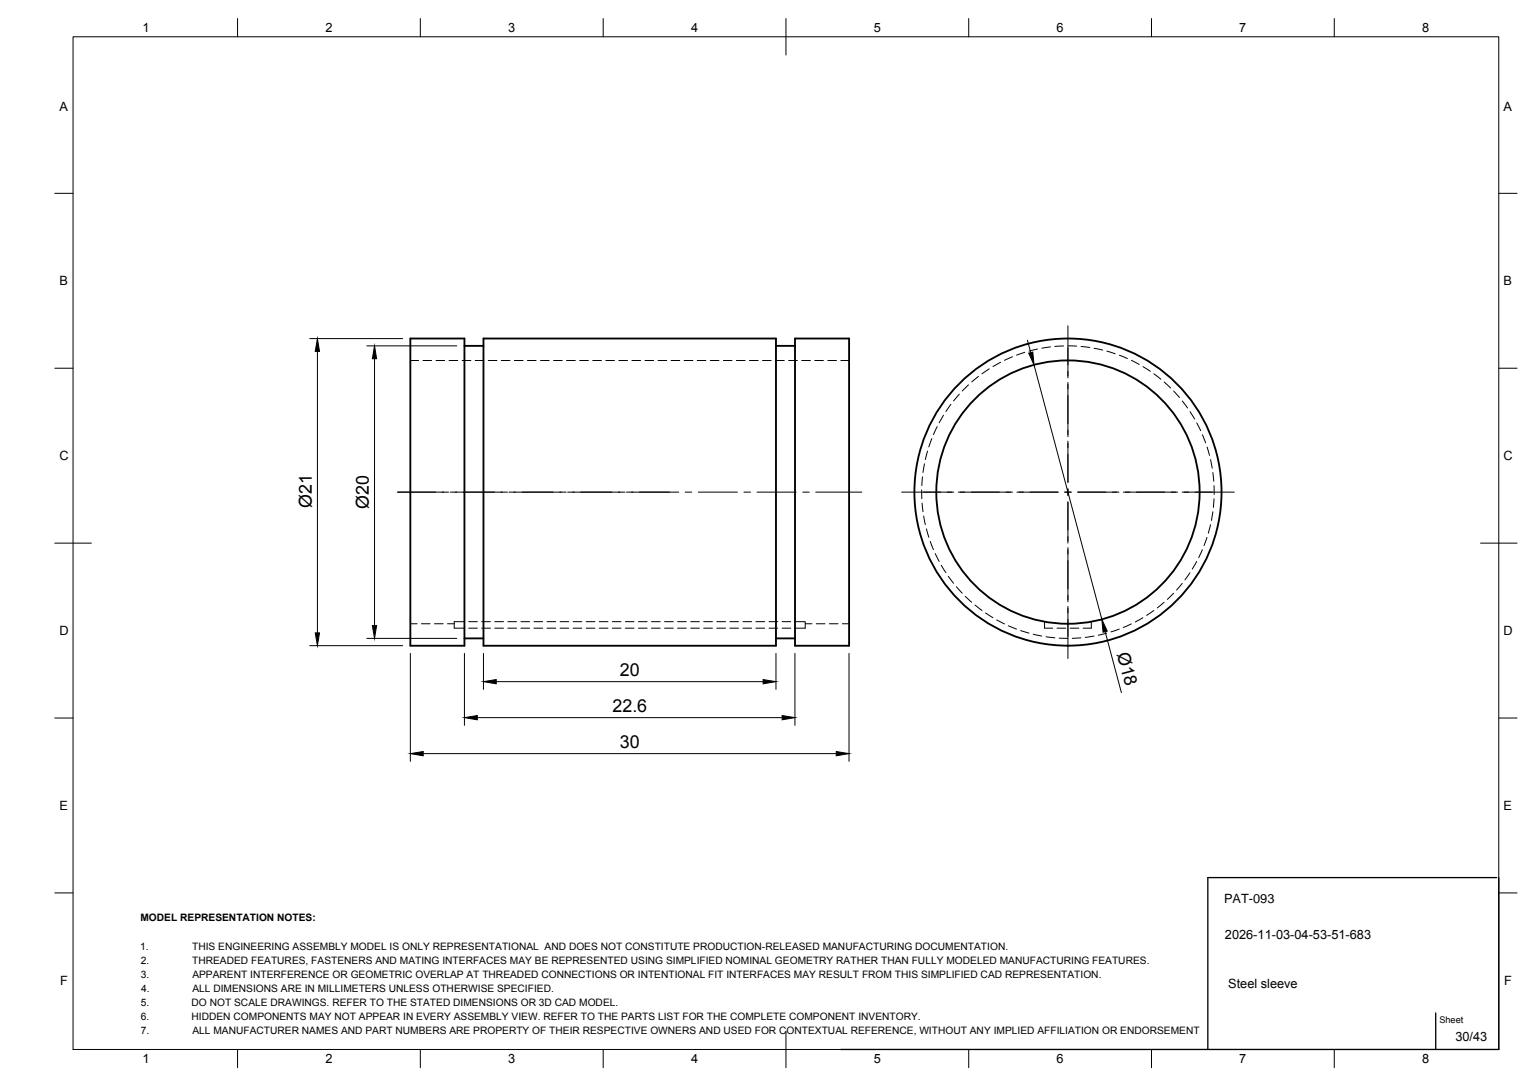
ISO-10303-21;
HEADER;
/* Generated by software containing ST-Developer
 * from STEP Tools, Inc. (www.steptools.com) 
 */

FILE_DESCRIPTION(
/* description */ ('Self-centering screw clamp'),
/* implementation_level */ '2;1');

FILE_NAME(
/* name */ 'Steel sleeve.step',
/* time_stamp */ '2026-10-28T03:25:31-07:00',
/* author */ (''),
/* organization */ (''),
/* preprocessor_version */ 'ST-DEVELOPER v20.2',
/* originating_system */ 'Autodesk Translation Framework v15.17.0.0',
/* authorisation */ '');

FILE_SCHEMA (('AUTOMOTIVE_DESIGN { 1 0 10303 214 3 1 1 }'));
ENDSEC;

DATA;
#10=MECHANICAL_DESIGN_GEOMETRIC_PRESENTATION_REPRESENTATION('',(#660),#16799);
#571=SHAPE_REPRESENTATION_RELATIONSHIP('SRR','None',#17048,#612);
#612=ADVANCED_BREP_SHAPE_REPRESENTATION('',(#708),#16786);
#660=STYLED_ITEM('',(#17340),#708);
#708=MANIFOLD_SOLID_BREP('Body1',#9111);
#981=FACE_BOUND('',#2433,.T.);
#982=FACE_BOUND('',#2436,.T.);
#983=FACE_BOUND('',#2439,.T.);
#984=FACE_BOUND('',#2442,.T.);
#985=FACE_BOUND('',#2445,.T.);
#986=FACE_BOUND('',#2448,.T.);
#987=FACE_BOUND('',#2450,.T.);
#1200=PLANE('',#10430);
#1201=PLANE('',#10432);
#1202=PLANE('',#10433);
#1203=PLANE('',#10435);
#1204=PLANE('',#10436);
#1205=PLANE('',#10437);
#1206=PLANE('',#10442);
#1207=PLANE('',#10446);
#1208=PLANE('',#10450);
#1209=PLANE('',#10454);
#1210=PLANE('',#10458);
#1660=FACE_OUTER_BOUND('',#2427,.T.);
#1661=FACE_OUTER_BOUND('',#2428,.T.);
#1662=FACE_OUTER_BOUND('',#2429,.T.);
#1663=FACE_OUTER_BOUND('',#2430,.T.);
#1664=FACE_OUTER_BOUND('',#2431,.T.);
#1665=FACE_OUTER_BOUND('',#2432,.T.);
#1666=FACE_OUTER_BOUND('',#2434,.T.);
#1667=FACE_OUTER_BOUND('',#2435,.T.);
#1668=FACE_OUTER_BOUND('',#2437,.T.);
#1669=FACE_OUTER_BOUND('',#2438,.T.);
#1670=FACE_OUTER_BOUND('',#2440,.T.);
#1671=FACE_OUTER_BOUND('',#2441,.T.);
#1672=FACE_OUTER_BOUND('',#2443,.T.);
#1673=FACE_OUTER_BOUND('',#2444,.T.);
#1674=FACE_OUTER_BOUND('',#2446,.T.);
#1675=FACE_OUTER_BOUND('',#2447,.T.);
#1676=FACE_OUTER_BOUND('',#2449,.T.);
#2427=EDGE_LOOP('',(#7911,#7912,#7913,#7914));
#2428=EDGE_LOOP('',(#7915,#7916,#7917,#7918));
#2429=EDGE_LOOP('',(#7919,#7920,#7921,#7922));
#2430=EDGE_LOOP('',(#7923,#7924,#7925,#7926));
#2431=EDGE_LOOP('',(#7927,#7928,#7929,#7930));
#2432=EDGE_LOOP('',(#7931));
#2433=EDGE_LOOP('',(#7932));
#2434=EDGE_LOOP('',(#7933,#7934,#7935,#7936));
#2435=EDGE_LOOP('',(#7937));
#2436=EDGE_LOOP('',(#7938));
#2437=EDGE_LOOP('',(#7939,#7940,#7941,#7942));
#2438=EDGE_LOOP('',(#7943));
#2439=EDGE_LOOP('',(#7944));
#2440=EDGE_LOOP('',(#7945,#7946,#7947,#7948));
#2441=EDGE_LOOP('',(#7949));
#2442=EDGE_LOOP('',(#7950));
#2443=EDGE_LOOP('',(#7951,#7952,#7953,#7954));
#2444=EDGE_LOOP('',(#7955));
#2445=EDGE_LOOP('',(#7956));
#2446=EDGE_LOOP('',(#7957,#7958,#7959,#7960));
#2447=EDGE_LOOP('',(#7961));
#2448=EDGE_LOOP('',(#7962));
#2449=EDGE_LOOP('',(#7963,#7964,#7965,#7966));
#2450=EDGE_LOOP('',(#7967,#7968,#7969,#7970));
#3026=LINE('',#15984,#3599);
#3027=LINE('',#15986,#3600);
#3028=LINE('',#15987,#3601);
#3029=LINE('',#15990,#3602);
#3030=LINE('',#15992,#3603);
#3031=LINE('',#15993,#3604);
#3032=LINE('',#15998,#3605);
#3033=LINE('',#15999,#3606);
#3034=LINE('',#16001,#3607);
#3035=LINE('',#16002,#3608);
#3036=LINE('',#16012,#3609);
#3037=LINE('',#16019,#3610);
#3038=LINE('',#16026,#3611);
#3039=LINE('',#16033,#3612);
#3040=LINE('',#16040,#3613);
#3041=LINE('',#16045,#3614);
#3599=VECTOR('',#12911,1.);
#3600=VECTOR('',#12912,1.);
#3601=VECTOR('',#12913,1.);
#3602=VECTOR('',#12916,1.);
#3603=VECTOR('',#12917,1.);
#3604=VECTOR('',#12918,1.);
#3605=VECTOR('',#12923,1.);
#3606=VECTOR('',#12924,1.);
#3607=VECTOR('',#12927,1.);
#3608=VECTOR('',#12928,1.);
#3609=VECTOR('',#12941,1.05);
#3610=VECTOR('',#12950,1.);
#3611=VECTOR('',#12959,1.05);
#3612=VECTOR('',#12968,1.);
#3613=VECTOR('',#12977,1.05);
#3614=VECTOR('',#12984,0.9);
#4148=CIRCLE('',#10431,0.9);
#4149=CIRCLE('',#10434,0.9);
#4150=CIRCLE('',#10438,1.05);
#4151=CIRCLE('',#10439,0.9);
#4152=CIRCLE('',#10441,1.05);
#4153=CIRCLE('',#10443,1.);
#4154=CIRCLE('',#10445,1.);
#4155=CIRCLE('',#10447,1.05);
#4156=CIRCLE('',#10449,1.05);
#4157=CIRCLE('',#10451,1.);
#4158=CIRCLE('',#10453,1.);
#4159=CIRCLE('',#10455,1.05);
#4160=CIRCLE('',#10457,1.05);
#4161=CIRCLE('',#10459,0.9);
#4831=VERTEX_POINT('',#15980);
#4832=VERTEX_POINT('',#15981);
#4833=VERTEX_POINT('',#15983);
#4834=VERTEX_POINT('',#15985);
#4835=VERTEX_POINT('',#15989);
#4836=VERTEX_POINT('',#15991);
#4837=VERTEX_POINT('',#15995);
#4838=VERTEX_POINT('',#15997);
#4839=VERTEX_POINT('',#16005);
#4840=VERTEX_POINT('',#16007);
#4841=VERTEX_POINT('',#16010);
#4842=VERTEX_POINT('',#16014);
#4843=VERTEX_POINT('',#16017);
#4844=VERTEX_POINT('',#16021);
#4845=VERTEX_POINT('',#16024);
#4846=VERTEX_POINT('',#16028);
#4847=VERTEX_POINT('',#16031);
#4848=VERTEX_POINT('',#16035);
#4849=VERTEX_POINT('',#16038);
#4850=VERTEX_POINT('',#16042);
#5880=EDGE_CURVE('',#4831,#4832,#4148,.T.);
#5881=EDGE_CURVE('',#4833,#4831,#3026,.T.);
#5882=EDGE_CURVE('',#4834,#4833,#3027,.T.);
#5883=EDGE_CURVE('',#4832,#4834,#3028,.T.);
#5884=EDGE_CURVE('',#4832,#4835,#3029,.T.);
#5885=EDGE_CURVE('',#4836,#4834,#3030,.T.);
#5886=EDGE_CURVE('',#4836,#4835,#3031,.T.);
#5887=EDGE_CURVE('',#4835,#4837,#4149,.T.);
#5888=EDGE_CURVE('',#4838,#4836,#3032,.T.);
#5889=EDGE_CURVE('',#4837,#4838,#3033,.T.);
#5890=EDGE_CURVE('',#4837,#4831,#3034,.T.);
#5891=EDGE_CURVE('',#4838,#4833,#3035,.T.);
#5892=EDGE_CURVE('',#4839,#4839,#4150,.T.);
#5893=EDGE_CURVE('',#4840,#4840,#4151,.T.);
#5894=EDGE_CURVE('',#4841,#4841,#4152,.T.);
#5895=EDGE_CURVE('',#4841,#4839,#3036,.T.);
#5896=EDGE_CURVE('',#4842,#4842,#4153,.T.);
#5897=EDGE_CURVE('',#4843,#4843,#4154,.T.);
#5898=EDGE_CURVE('',#4843,#4842,#3037,.T.);
#5899=EDGE_CURVE('',#4844,#4844,#4155,.T.);
#5900=EDGE_CURVE('',#4845,#4845,#4156,.T.);
#5901=EDGE_CURVE('',#4845,#4844,#3038,.T.);
#5902=EDGE_CURVE('',#4846,#4846,#4157,.T.);
#5903=EDGE_CURVE('',#4847,#4847,#4158,.T.);
#5904=EDGE_CURVE('',#4847,#4846,#3039,.T.);
#5905=EDGE_CURVE('',#4848,#4848,#4159,.T.);
#5906=EDGE_CURVE('',#4849,#4849,#4160,.T.);
#5907=EDGE_CURVE('',#4849,#4848,#3040,.T.);
#5908=EDGE_CURVE('',#4850,#4850,#4161,.T.);
#5909=EDGE_CURVE('',#4850,#4840,#3041,.T.);
#7911=ORIENTED_EDGE('',*,*,#5880,.F.);
#7912=ORIENTED_EDGE('',*,*,#5881,.F.);
#7913=ORIENTED_EDGE('',*,*,#5882,.F.);
#7914=ORIENTED_EDGE('',*,*,#5883,.F.);
#7915=ORIENTED_EDGE('',*,*,#5884,.F.);
#7916=ORIENTED_EDGE('',*,*,#5883,.T.);
#7917=ORIENTED_EDGE('',*,*,#5885,.F.);
#7918=ORIENTED_EDGE('',*,*,#5886,.T.);
#7919=ORIENTED_EDGE('',*,*,#5887,.F.);
#7920=ORIENTED_EDGE('',*,*,#5886,.F.);
#7921=ORIENTED_EDGE('',*,*,#5888,.F.);
#7922=ORIENTED_EDGE('',*,*,#5889,.F.);
#7923=ORIENTED_EDGE('',*,*,#5890,.F.);
#7924=ORIENTED_EDGE('',*,*,#5889,.T.);
#7925=ORIENTED_EDGE('',*,*,#5891,.T.);
#7926=ORIENTED_EDGE('',*,*,#5881,.T.);
#7927=ORIENTED_EDGE('',*,*,#5891,.F.);
#7928=ORIENTED_EDGE('',*,*,#5888,.T.);
#7929=ORIENTED_EDGE('',*,*,#5885,.T.);
#7930=ORIENTED_EDGE('',*,*,#5882,.T.);
#7931=ORIENTED_EDGE('',*,*,#5892,.F.);
#7932=ORIENTED_EDGE('',*,*,#5893,.T.);
#7933=ORIENTED_EDGE('',*,*,#5894,.F.);
#7934=ORIENTED_EDGE('',*,*,#5895,.T.);
#7935=ORIENTED_EDGE('',*,*,#5892,.T.);
#7936=ORIENTED_EDGE('',*,*,#5895,.F.);
#7937=ORIENTED_EDGE('',*,*,#5894,.T.);
#7938=ORIENTED_EDGE('',*,*,#5896,.F.);
#7939=ORIENTED_EDGE('',*,*,#5897,.F.);
#7940=ORIENTED_EDGE('',*,*,#5898,.T.);
#7941=ORIENTED_EDGE('',*,*,#5896,.T.);
#7942=ORIENTED_EDGE('',*,*,#5898,.F.);
#7943=ORIENTED_EDGE('',*,*,#5899,.F.);
#7944=ORIENTED_EDGE('',*,*,#5897,.T.);
#7945=ORIENTED_EDGE('',*,*,#5900,.F.);
#7946=ORIENTED_EDGE('',*,*,#5901,.T.);
#7947=ORIENTED_EDGE('',*,*,#5899,.T.);
#7948=ORIENTED_EDGE('',*,*,#5901,.F.);
#7949=ORIENTED_EDGE('',*,*,#5900,.T.);
#7950=ORIENTED_EDGE('',*,*,#5902,.F.);
#7951=ORIENTED_EDGE('',*,*,#5903,.F.);
#7952=ORIENTED_EDGE('',*,*,#5904,.T.);
#7953=ORIENTED_EDGE('',*,*,#5902,.T.);
#7954=ORIENTED_EDGE('',*,*,#5904,.F.);
#7955=ORIENTED_EDGE('',*,*,#5905,.F.);
#7956=ORIENTED_EDGE('',*,*,#5903,.T.);
#7957=ORIENTED_EDGE('',*,*,#5906,.F.);
#7958=ORIENTED_EDGE('',*,*,#5907,.T.);
#7959=ORIENTED_EDGE('',*,*,#5905,.T.);
#7960=ORIENTED_EDGE('',*,*,#5907,.F.);
#7961=ORIENTED_EDGE('',*,*,#5906,.T.);
#7962=ORIENTED_EDGE('',*,*,#5908,.F.);
#7963=ORIENTED_EDGE('',*,*,#5908,.T.);
#7964=ORIENTED_EDGE('',*,*,#5909,.T.);
#7965=ORIENTED_EDGE('',*,*,#5893,.F.);
#7966=ORIENTED_EDGE('',*,*,#5909,.F.);
#7967=ORIENTED_EDGE('',*,*,#5887,.T.);
#7968=ORIENTED_EDGE('',*,*,#5890,.T.);
#7969=ORIENTED_EDGE('',*,*,#5880,.T.);
#7970=ORIENTED_EDGE('',*,*,#5884,.T.);
#8536=CYLINDRICAL_SURFACE('',#10440,1.05);
#8537=CYLINDRICAL_SURFACE('',#10444,1.);
#8538=CYLINDRICAL_SURFACE('',#10448,1.05);
#8539=CYLINDRICAL_SURFACE('',#10452,1.);
#8540=CYLINDRICAL_SURFACE('',#10456,1.05);
#8541=CYLINDRICAL_SURFACE('',#10460,0.9);
#8958=ADVANCED_FACE('',(#1660),#1200,.F.);
#8959=ADVANCED_FACE('',(#1661),#1201,.F.);
#8960=ADVANCED_FACE('',(#1662),#1202,.F.);
#8961=ADVANCED_FACE('',(#1663),#1203,.F.);
#8962=ADVANCED_FACE('',(#1664),#1204,.F.);
#8963=ADVANCED_FACE('',(#1665,#981),#1205,.T.);
#8964=ADVANCED_FACE('',(#1666),#8536,.T.);
#8965=ADVANCED_FACE('',(#1667,#982),#1206,.T.);
#8966=ADVANCED_FACE('',(#1668),#8537,.T.);
#8967=ADVANCED_FACE('',(#1669,#983),#1207,.T.);
#8968=ADVANCED_FACE('',(#1670),#8538,.T.);
#8969=ADVANCED_FACE('',(#1671,#984),#1208,.T.);
#8970=ADVANCED_FACE('',(#1672),#8539,.T.);
#8971=ADVANCED_FACE('',(#1673,#985),#1209,.T.);
#8972=ADVANCED_FACE('',(#1674),#8540,.T.);
#8973=ADVANCED_FACE('',(#1675,#986),#1210,.T.);
#8974=ADVANCED_FACE('',(#1676,#987),#8541,.F.);
#9111=CLOSED_SHELL('',(#8958,#8959,#8960,#8961,#8962,#8963,#8964,#8965,
#8966,#8967,#8968,#8969,#8970,#8971,#8972,#8973,#8974));
#10429=AXIS2_PLACEMENT_3D('',#15978,#12905,#12906);
#10430=AXIS2_PLACEMENT_3D('',#15979,#12907,#12908);
#10431=AXIS2_PLACEMENT_3D('',#15982,#12909,#12910);
#10432=AXIS2_PLACEMENT_3D('',#15988,#12914,#12915);
#10433=AXIS2_PLACEMENT_3D('',#15994,#12919,#12920);
#10434=AXIS2_PLACEMENT_3D('',#15996,#12921,#12922);
#10435=AXIS2_PLACEMENT_3D('',#16000,#12925,#12926);
#10436=AXIS2_PLACEMENT_3D('',#16003,#12929,#12930);
#10437=AXIS2_PLACEMENT_3D('',#16004,#12931,#12932);
#10438=AXIS2_PLACEMENT_3D('',#16006,#12933,#12934);
#10439=AXIS2_PLACEMENT_3D('',#16008,#12935,#12936);
#10440=AXIS2_PLACEMENT_3D('',#16009,#12937,#12938);
#10441=AXIS2_PLACEMENT_3D('',#16011,#12939,#12940);
#10442=AXIS2_PLACEMENT_3D('',#16013,#12942,#12943);
#10443=AXIS2_PLACEMENT_3D('',#16015,#12944,#12945);
#10444=AXIS2_PLACEMENT_3D('',#16016,#12946,#12947);
#10445=AXIS2_PLACEMENT_3D('',#16018,#12948,#12949);
#10446=AXIS2_PLACEMENT_3D('',#16020,#12951,#12952);
#10447=AXIS2_PLACEMENT_3D('',#16022,#12953,#12954);
#10448=AXIS2_PLACEMENT_3D('',#16023,#12955,#12956);
#10449=AXIS2_PLACEMENT_3D('',#16025,#12957,#12958);
#10450=AXIS2_PLACEMENT_3D('',#16027,#12960,#12961);
#10451=AXIS2_PLACEMENT_3D('',#16029,#12962,#12963);
#10452=AXIS2_PLACEMENT_3D('',#16030,#12964,#12965);
#10453=AXIS2_PLACEMENT_3D('',#16032,#12966,#12967);
#10454=AXIS2_PLACEMENT_3D('',#16034,#12969,#12970);
#10455=AXIS2_PLACEMENT_3D('',#16036,#12971,#12972);
#10456=AXIS2_PLACEMENT_3D('',#16037,#12973,#12974);
#10457=AXIS2_PLACEMENT_3D('',#16039,#12975,#12976);
#10458=AXIS2_PLACEMENT_3D('',#16041,#12978,#12979);
#10459=AXIS2_PLACEMENT_3D('',#16043,#12980,#12981);
#10460=AXIS2_PLACEMENT_3D('',#16044,#12982,#12983);
#12905=DIRECTION('axis',(0.,0.,1.));
#12906=DIRECTION('refdir',(1.,0.,0.));
#12907=DIRECTION('center_axis',(0.,1.,0.));
#12908=DIRECTION('ref_axis',(0.,0.,1.));
#12909=DIRECTION('center_axis',(0.,-1.,0.));
#12910=DIRECTION('ref_axis',(1.,0.,0.));
#12911=DIRECTION('',(-1.,0.,0.));
#12912=DIRECTION('',(0.,0.,-1.));
#12913=DIRECTION('',(1.,0.,0.));
#12914=DIRECTION('center_axis',(0.,0.,1.));
#12915=DIRECTION('ref_axis',(1.,0.,0.));
#12916=DIRECTION('',(0.,-1.,0.));
#12917=DIRECTION('',(0.,1.,0.));
#12918=DIRECTION('',(-1.,0.,0.));
#12919=DIRECTION('center_axis',(0.,-1.,0.));
#12920=DIRECTION('ref_axis',(0.,0.,-1.));
#12921=DIRECTION('center_axis',(0.,1.,0.));
#12922=DIRECTION('ref_axis',(1.,0.,0.));
#12923=DIRECTION('',(0.,0.,1.));
#12924=DIRECTION('',(1.,0.,0.));
#12925=DIRECTION('center_axis',(0.,0.,-1.));
#12926=DIRECTION('ref_axis',(-1.,0.,0.));
#12927=DIRECTION('',(0.,1.,0.));
#12928=DIRECTION('',(0.,1.,0.));
#12929=DIRECTION('center_axis',(1.,0.,0.));
#12930=DIRECTION('ref_axis',(0.,0.,-1.));
#12931=DIRECTION('center_axis',(0.,1.,0.));
#12932=DIRECTION('ref_axis',(0.,0.,1.));
#12933=DIRECTION('center_axis',(0.,-1.,0.));
#12934=DIRECTION('ref_axis',(1.,0.,0.));
#12935=DIRECTION('center_axis',(0.,-1.,0.));
#12936=DIRECTION('ref_axis',(1.,0.,0.));
#12937=DIRECTION('center_axis',(0.,-1.,0.));
#12938=DIRECTION('ref_axis',(1.,0.,0.));
#12939=DIRECTION('center_axis',(0.,-1.,0.));
#12940=DIRECTION('ref_axis',(1.,0.,0.));
#12941=DIRECTION('',(0.,1.,0.));
#12942=DIRECTION('center_axis',(0.,-1.,0.));
#12943=DIRECTION('ref_axis',(0.,0.,-1.));
#12944=DIRECTION('center_axis',(0.,-1.,0.));
#12945=DIRECTION('ref_axis',(1.,0.,0.));
#12946=DIRECTION('center_axis',(0.,-1.,0.));
#12947=DIRECTION('ref_axis',(1.,0.,0.));
#12948=DIRECTION('center_axis',(0.,-1.,0.));
#12949=DIRECTION('ref_axis',(1.,0.,0.));
#12950=DIRECTION('',(0.,1.,0.));
#12951=DIRECTION('center_axis',(0.,1.,0.));
#12952=DIRECTION('ref_axis',(0.,0.,1.));
#12953=DIRECTION('center_axis',(0.,-1.,0.));
#12954=DIRECTION('ref_axis',(1.,0.,0.));
#12955=DIRECTION('center_axis',(0.,-1.,0.));
#12956=DIRECTION('ref_axis',(1.,0.,0.));
#12957=DIRECTION('center_axis',(0.,-1.,0.));
#12958=DIRECTION('ref_axis',(1.,0.,0.));
#12959=DIRECTION('',(0.,1.,0.));
#12960=DIRECTION('center_axis',(0.,-1.,0.));
#12961=DIRECTION('ref_axis',(0.,0.,-1.));
#12962=DIRECTION('center_axis',(0.,-1.,0.));
#12963=DIRECTION('ref_axis',(1.,0.,0.));
#12964=DIRECTION('center_axis',(0.,-1.,0.));
#12965=DIRECTION('ref_axis',(1.,0.,0.));
#12966=DIRECTION('center_axis',(0.,-1.,0.));
#12967=DIRECTION('ref_axis',(1.,0.,0.));
#12968=DIRECTION('',(0.,1.,0.));
#12969=DIRECTION('center_axis',(0.,1.,0.));
#12970=DIRECTION('ref_axis',(0.,0.,1.));
#12971=DIRECTION('center_axis',(0.,-1.,0.));
#12972=DIRECTION('ref_axis',(1.,0.,0.));
#12973=DIRECTION('center_axis',(0.,-1.,0.));
#12974=DIRECTION('ref_axis',(1.,0.,0.));
#12975=DIRECTION('center_axis',(0.,-1.,0.));
#12976=DIRECTION('ref_axis',(1.,0.,0.));
#12977=DIRECTION('',(0.,1.,0.));
#12978=DIRECTION('center_axis',(0.,-1.,0.));
#12979=DIRECTION('ref_axis',(0.,0.,-1.));
#12980=DIRECTION('center_axis',(0.,-1.,0.));
#12981=DIRECTION('ref_axis',(1.,0.,0.));
#12982=DIRECTION('center_axis',(0.,-1.,0.));
#12983=DIRECTION('ref_axis',(1.,0.,0.));
#12984=DIRECTION('',(0.,1.,0.));
#15978=CARTESIAN_POINT('',(0.,0.,0.));
#15979=CARTESIAN_POINT('Origin',(0.75,1.2,0.));
#15980=CARTESIAN_POINT('',(0.885663593019381,1.2,-0.16));
#15981=CARTESIAN_POINT('',(0.885663593019381,1.2,0.16));
#15982=CARTESIAN_POINT('Origin',(0.,1.2,0.));
#15983=CARTESIAN_POINT('',(0.93,1.2,-0.16));
#15984=CARTESIAN_POINT('',(0.93,1.2,-0.16));
#15985=CARTESIAN_POINT('',(0.93,1.2,0.16));
#15986=CARTESIAN_POINT('',(0.93,1.2,0.16));
#15987=CARTESIAN_POINT('',(0.57,1.2,0.16));
#15988=CARTESIAN_POINT('Origin',(0.57,0.,0.16));
#15989=CARTESIAN_POINT('',(0.885663593019381,-1.2,0.16));
#15990=CARTESIAN_POINT('',(0.885663593019381,0.,0.16));
#15991=CARTESIAN_POINT('',(0.93,-1.2,0.16));
#15992=CARTESIAN_POINT('',(0.93,0.,0.16));
#15993=CARTESIAN_POINT('',(0.57,-1.2,0.16));
#15994=CARTESIAN_POINT('Origin',(0.75,-1.2,0.));
#15995=CARTESIAN_POINT('',(0.885663593019381,-1.2,-0.16));
#15996=CARTESIAN_POINT('Origin',(0.,-1.2,0.));
#15997=CARTESIAN_POINT('',(0.93,-1.2,-0.16));
#15998=CARTESIAN_POINT('',(0.93,-1.2,0.16));
#15999=CARTESIAN_POINT('',(0.93,-1.2,-0.16));
#16000=CARTESIAN_POINT('Origin',(0.93,0.,-0.16));
#16001=CARTESIAN_POINT('',(0.885663593019381,0.,-0.16));
#16002=CARTESIAN_POINT('',(0.93,0.,-0.16));
#16003=CARTESIAN_POINT('Origin',(0.93,0.,0.16));
#16004=CARTESIAN_POINT('Origin',(1.05,1.5,0.));
#16005=CARTESIAN_POINT('',(-1.05,1.5,-1.28587913910472E-16));
#16006=CARTESIAN_POINT('Origin',(0.,1.5,0.));
#16007=CARTESIAN_POINT('',(-0.9,1.5,-1.10218211923262E-16));
#16008=CARTESIAN_POINT('Origin',(0.,1.5,0.));
#16009=CARTESIAN_POINT('Origin',(0.,1.315,0.));
#16010=CARTESIAN_POINT('',(-1.05,1.13,-1.28587913910472E-16));
#16011=CARTESIAN_POINT('Origin',(0.,1.13,0.));
#16012=CARTESIAN_POINT('',(-1.05,1.315,-1.28587913910472E-16));
#16013=CARTESIAN_POINT('Origin',(1.,1.13,0.));
#16014=CARTESIAN_POINT('',(-1.,1.13,-1.22464679914735E-16));
#16015=CARTESIAN_POINT('Origin',(0.,1.13,0.));
#16016=CARTESIAN_POINT('Origin',(0.,1.065,0.));
#16017=CARTESIAN_POINT('',(-1.,1.,-1.22464679914735E-16));
#16018=CARTESIAN_POINT('Origin',(0.,1.,0.));
#16019=CARTESIAN_POINT('',(-1.,1.065,-1.22464679914735E-16));
#16020=CARTESIAN_POINT('Origin',(1.05,1.,0.));
#16021=CARTESIAN_POINT('',(-1.05,1.,-1.28587913910472E-16));
#16022=CARTESIAN_POINT('Origin',(0.,1.,0.));
#16023=CARTESIAN_POINT('Origin',(0.,0.,0.));
#16024=CARTESIAN_POINT('',(-1.05,-1.,-1.28587913910472E-16));
#16025=CARTESIAN_POINT('Origin',(0.,-1.,0.));
#16026=CARTESIAN_POINT('',(-1.05,0.,-1.28587913910472E-16));
#16027=CARTESIAN_POINT('Origin',(1.,-1.,0.));
#16028=CARTESIAN_POINT('',(-1.,-1.,-1.22464679914735E-16));
#16029=CARTESIAN_POINT('Origin',(0.,-1.,0.));
#16030=CARTESIAN_POINT('Origin',(0.,-1.065,0.));
#16031=CARTESIAN_POINT('',(-1.,-1.13,-1.22464679914735E-16));
#16032=CARTESIAN_POINT('Origin',(0.,-1.13,0.));
#16033=CARTESIAN_POINT('',(-1.,-1.065,-1.22464679914735E-16));
#16034=CARTESIAN_POINT('Origin',(1.05,-1.13,0.));
#16035=CARTESIAN_POINT('',(-1.05,-1.13,-1.28587913910472E-16));
#16036=CARTESIAN_POINT('Origin',(0.,-1.13,0.));
#16037=CARTESIAN_POINT('Origin',(0.,-1.315,0.));
#16038=CARTESIAN_POINT('',(-1.05,-1.5,-1.28587913910472E-16));
#16039=CARTESIAN_POINT('Origin',(0.,-1.5,0.));
#16040=CARTESIAN_POINT('',(-1.05,-1.315,-1.28587913910472E-16));
#16041=CARTESIAN_POINT('Origin',(0.9,-1.5,0.));
#16042=CARTESIAN_POINT('',(-0.9,-1.5,-1.10218211923262E-16));
#16043=CARTESIAN_POINT('Origin',(0.,-1.5,0.));
#16044=CARTESIAN_POINT('Origin',(0.,0.,0.));
#16045=CARTESIAN_POINT('',(-0.9,0.,-1.10218211923262E-16));
#16737=UNCERTAINTY_MEASURE_WITH_UNIT(LENGTH_MEASURE(0.001),#16800,
'DISTANCE_ACCURACY_VALUE',
'Maximum model space distance between geometric entities at asserted c
onnectivities');
#16750=UNCERTAINTY_MEASURE_WITH_UNIT(LENGTH_MEASURE(0.001),#16800,
'DISTANCE_ACCURACY_VALUE',
'Maximum model space distance between geometric entities at asserted c
onnectivities');
#16786=(
GEOMETRIC_REPRESENTATION_CONTEXT(3)
GLOBAL_UNCERTAINTY_ASSIGNED_CONTEXT((#16737))
GLOBAL_UNIT_ASSIGNED_CONTEXT((#16800,#16802,#16803))
REPRESENTATION_CONTEXT('','3D')
);
#16799=(
GEOMETRIC_REPRESENTATION_CONTEXT(3)
GLOBAL_UNCERTAINTY_ASSIGNED_CONTEXT((#16750))
GLOBAL_UNIT_ASSIGNED_CONTEXT((#16800,#16802,#16803))
REPRESENTATION_CONTEXT('','3D')
);
#16800=(
LENGTH_UNIT()
NAMED_UNIT(*)
SI_UNIT(.CENTI.,.METRE.)
);
#16802=(
NAMED_UNIT(*)
PLANE_ANGLE_UNIT()
SI_UNIT($,.RADIAN.)
);
#16803=(
NAMED_UNIT(*)
SI_UNIT($,.STERADIAN.)
SOLID_ANGLE_UNIT()
);
#16839=SHAPE_DEFINITION_REPRESENTATION(#16892,#17048);
#16892=PRODUCT_DEFINITION_SHAPE('',$,#17097);
#17048=SHAPE_REPRESENTATION('',(#10429),#16786);
#17061=PRODUCT_DEFINITION_CONTEXT('part definition',#17207,'design');
#17097=PRODUCT_DEFINITION('Steel sleeve','Steel sleeve',#17145,#17061);
#17145=PRODUCT_DEFINITION_FORMATION('',$,#17244);
#17207=APPLICATION_CONTEXT(
'Core Data for Automotive Mechanical Design Process');
#17208=PRODUCT_CONTEXT('part definition',#17207,'mechanical');
#17244=PRODUCT('Steel sleeve','Steel sleeve','Steel sleeve',(#17208));
#17334=COLOUR_RGB('Off White',0.89,0.88,0.83);
#17335=FILL_AREA_STYLE_COLOUR('',#17334);
#17336=FILL_AREA_STYLE('',(#17335));
#17337=SURFACE_STYLE_FILL_AREA(#17336);
#17338=SURFACE_SIDE_STYLE('',(#17337));
#17339=SURFACE_STYLE_USAGE(.BOTH.,#17338);
#17340=PRESENTATION_STYLE_ASSIGNMENT((#17339));
ENDSEC;
END-ISO-10303-21;
